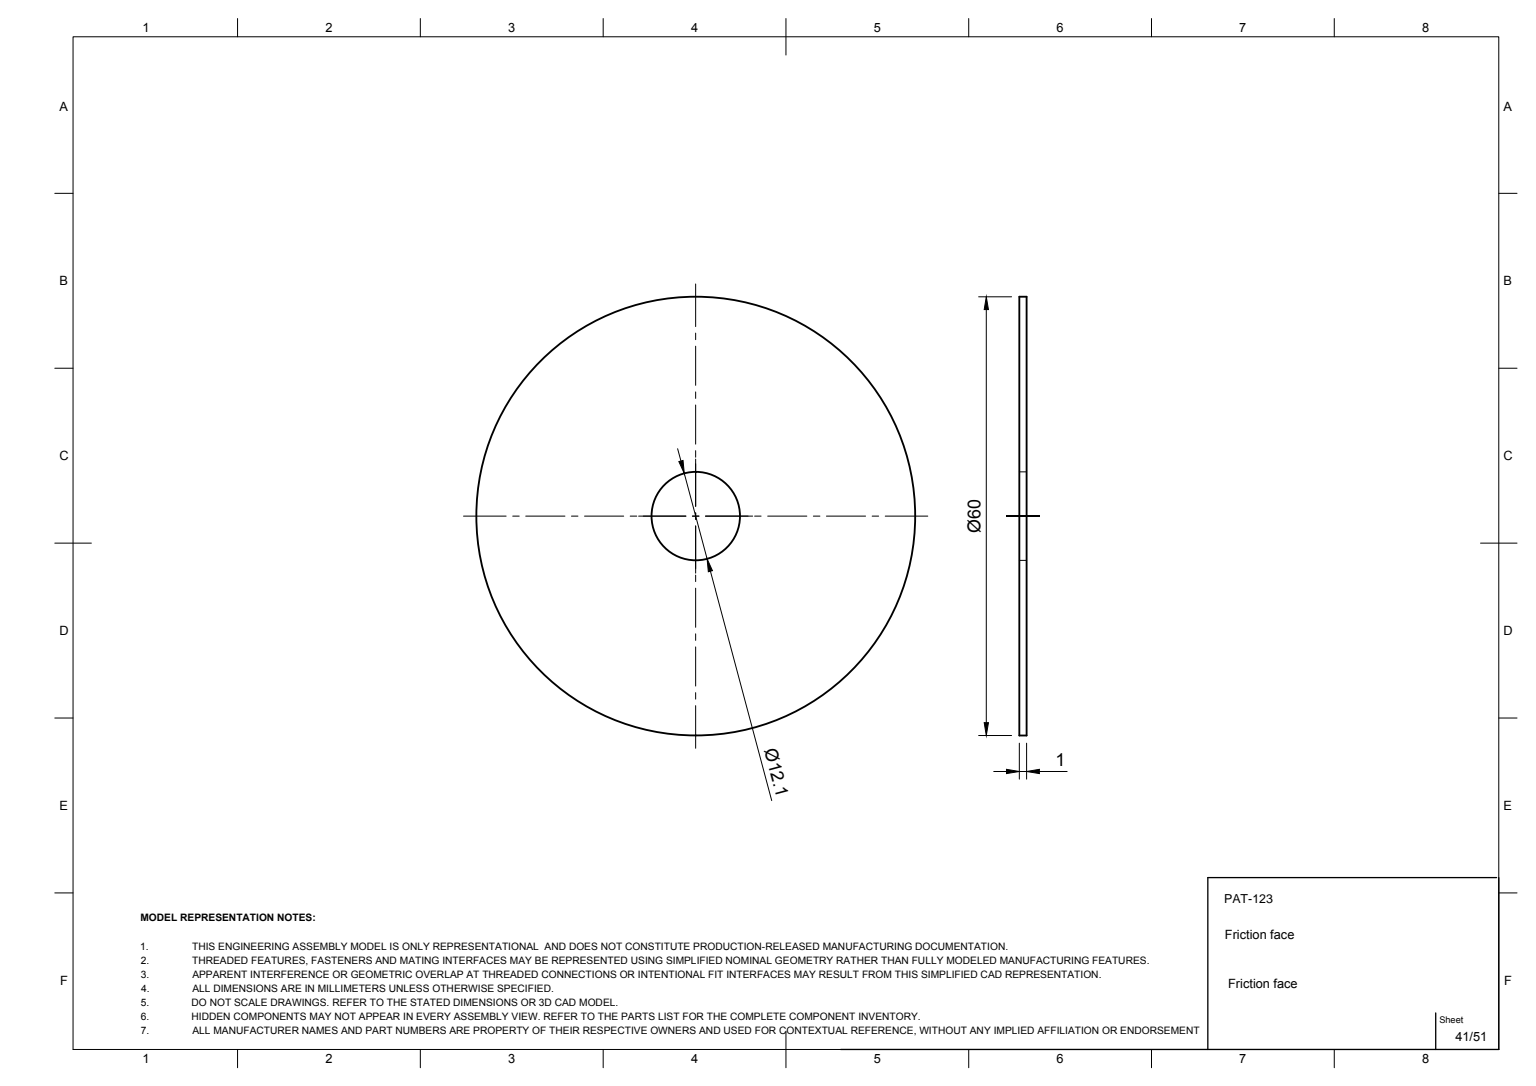
ISO-10303-21;
HEADER;
/* Generated by software containing ST-Developer
 * from STEP Tools, Inc. (www.steptools.com) 
 */

FILE_DESCRIPTION(
/* description */ ('Worm-less right-angle friction wheel drive'),
/* implementation_level */ '2;1');

FILE_NAME(
/* name */ 'Friction face.step',
/* time_stamp */ '2026-10-28T03:22:36-07:00',
/* author */ (''),
/* organization */ (''),
/* preprocessor_version */ 'ST-DEVELOPER v20.2',
/* originating_system */ 'Autodesk Translation Framework v15.17.0.0',
/* authorisation */ '');

FILE_SCHEMA (('AUTOMOTIVE_DESIGN { 1 0 10303 214 3 1 1 }'));
ENDSEC;

DATA;
#10=MECHANICAL_DESIGN_GEOMETRIC_PRESENTATION_REPRESENTATION('',(#654),#17046);
#553=SHAPE_REPRESENTATION_RELATIONSHIP('SRR','None',#17298,#600);
#600=ADVANCED_BREP_SHAPE_REPRESENTATION('',(#705),#17034);
#654=STYLED_ITEM('',(#17577),#705);
#705=MANIFOLD_SOLID_BREP('Body1',#8212);
#932=FACE_BOUND('',#2271,.T.);
#933=FACE_BOUND('',#2273,.T.);
#1147=PLANE('',#9528);
#1148=PLANE('',#9529);
#1585=FACE_OUTER_BOUND('',#2268,.T.);
#1586=FACE_OUTER_BOUND('',#2269,.T.);
#1587=FACE_OUTER_BOUND('',#2270,.T.);
#1588=FACE_OUTER_BOUND('',#2272,.T.);
#2268=EDGE_LOOP('',(#7166,#7167,#7168,#7169));
#2269=EDGE_LOOP('',(#7170,#7171,#7172,#7173));
#2270=EDGE_LOOP('',(#7174));
#2271=EDGE_LOOP('',(#7175));
#2272=EDGE_LOOP('',(#7176));
#2273=EDGE_LOOP('',(#7177));
#2802=LINE('',#16336,#3342);
#2803=LINE('',#16342,#3343);
#3342=VECTOR('',#11762,0.605);
#3343=VECTOR('',#11769,3.);
#3816=CIRCLE('',#9523,0.605);
#3817=CIRCLE('',#9524,0.605);
#3818=CIRCLE('',#9526,3.);
#3819=CIRCLE('',#9527,3.);
#4417=VERTEX_POINT('',#16333);
#4418=VERTEX_POINT('',#16335);
#4419=VERTEX_POINT('',#16339);
#4420=VERTEX_POINT('',#16341);
#5352=EDGE_CURVE('',#4417,#4417,#3816,.T.);
#5353=EDGE_CURVE('',#4417,#4418,#2802,.T.);
#5354=EDGE_CURVE('',#4418,#4418,#3817,.T.);
#5355=EDGE_CURVE('',#4419,#4419,#3818,.T.);
#5356=EDGE_CURVE('',#4419,#4420,#2803,.T.);
#5357=EDGE_CURVE('',#4420,#4420,#3819,.T.);
#7166=ORIENTED_EDGE('',*,*,#5352,.F.);
#7167=ORIENTED_EDGE('',*,*,#5353,.T.);
#7168=ORIENTED_EDGE('',*,*,#5354,.T.);
#7169=ORIENTED_EDGE('',*,*,#5353,.F.);
#7170=ORIENTED_EDGE('',*,*,#5355,.F.);
#7171=ORIENTED_EDGE('',*,*,#5356,.T.);
#7172=ORIENTED_EDGE('',*,*,#5357,.T.);
#7173=ORIENTED_EDGE('',*,*,#5356,.F.);
#7174=ORIENTED_EDGE('',*,*,#5355,.T.);
#7175=ORIENTED_EDGE('',*,*,#5352,.T.);
#7176=ORIENTED_EDGE('',*,*,#5357,.F.);
#7177=ORIENTED_EDGE('',*,*,#5354,.F.);
#7677=CYLINDRICAL_SURFACE('',#9522,0.605);
#7678=CYLINDRICAL_SURFACE('',#9525,3.);
#8077=ADVANCED_FACE('',(#1585),#7677,.F.);
#8078=ADVANCED_FACE('',(#1586),#7678,.T.);
#8079=ADVANCED_FACE('',(#1587,#932),#1147,.T.);
#8080=ADVANCED_FACE('',(#1588,#933),#1148,.F.);
#8212=CLOSED_SHELL('',(#8077,#8078,#8079,#8080));
#9521=AXIS2_PLACEMENT_3D('',#16331,#11756,#11757);
#9522=AXIS2_PLACEMENT_3D('',#16332,#11758,#11759);
#9523=AXIS2_PLACEMENT_3D('',#16334,#11760,#11761);
#9524=AXIS2_PLACEMENT_3D('',#16337,#11763,#11764);
#9525=AXIS2_PLACEMENT_3D('',#16338,#11765,#11766);
#9526=AXIS2_PLACEMENT_3D('',#16340,#11767,#11768);
#9527=AXIS2_PLACEMENT_3D('',#16343,#11770,#11771);
#9528=AXIS2_PLACEMENT_3D('',#16344,#11772,#11773);
#9529=AXIS2_PLACEMENT_3D('',#16345,#11774,#11775);
#11756=DIRECTION('axis',(0.,0.,1.));
#11757=DIRECTION('refdir',(1.,0.,0.));
#11758=DIRECTION('center_axis',(0.,1.,0.));
#11759=DIRECTION('ref_axis',(1.,0.,0.));
#11760=DIRECTION('center_axis',(0.,-1.,0.));
#11761=DIRECTION('ref_axis',(1.,0.,0.));
#11762=DIRECTION('',(0.,-1.,0.));
#11763=DIRECTION('center_axis',(0.,-1.,0.));
#11764=DIRECTION('ref_axis',(1.,0.,0.));
#11765=DIRECTION('center_axis',(0.,1.,0.));
#11766=DIRECTION('ref_axis',(1.,0.,0.));
#11767=DIRECTION('center_axis',(0.,1.,0.));
#11768=DIRECTION('ref_axis',(1.,0.,0.));
#11769=DIRECTION('',(0.,-1.,0.));
#11770=DIRECTION('center_axis',(0.,1.,0.));
#11771=DIRECTION('ref_axis',(1.,0.,0.));
#11772=DIRECTION('center_axis',(0.,1.,0.));
#11773=DIRECTION('ref_axis',(1.,0.,0.));
#11774=DIRECTION('center_axis',(0.,1.,0.));
#11775=DIRECTION('ref_axis',(1.,0.,0.));
#16331=CARTESIAN_POINT('',(0.,0.,0.));
#16332=CARTESIAN_POINT('Origin',(0.,-0.1,7.));
#16333=CARTESIAN_POINT('',(-0.605,0.,7.));
#16334=CARTESIAN_POINT('Origin',(0.,0.,7.));
#16335=CARTESIAN_POINT('',(-0.605,-0.1,7.));
#16336=CARTESIAN_POINT('',(-0.605,-0.1,7.));
#16337=CARTESIAN_POINT('Origin',(0.,-0.1,7.));
#16338=CARTESIAN_POINT('Origin',(0.,-0.1,7.));
#16339=CARTESIAN_POINT('',(-3.,0.,7.));
#16340=CARTESIAN_POINT('Origin',(0.,0.,7.));
#16341=CARTESIAN_POINT('',(-3.,-0.1,7.));
#16342=CARTESIAN_POINT('',(-3.,-0.1,7.));
#16343=CARTESIAN_POINT('Origin',(0.,-0.1,7.));
#16344=CARTESIAN_POINT('Origin',(0.,0.,7.));
#16345=CARTESIAN_POINT('Origin',(0.,-0.1,7.));
#16981=UNCERTAINTY_MEASURE_WITH_UNIT(LENGTH_MEASURE(0.001),#17047,
'DISTANCE_ACCURACY_VALUE',
'Maximum model space distance between geometric entities at asserted c
onnectivities');
#16993=UNCERTAINTY_MEASURE_WITH_UNIT(LENGTH_MEASURE(0.001),#17047,
'DISTANCE_ACCURACY_VALUE',
'Maximum model space distance between geometric entities at asserted c
onnectivities');
#17034=(
GEOMETRIC_REPRESENTATION_CONTEXT(3)
GLOBAL_UNCERTAINTY_ASSIGNED_CONTEXT((#16981))
GLOBAL_UNIT_ASSIGNED_CONTEXT((#17047,#17049,#17050))
REPRESENTATION_CONTEXT('','3D')
);
#17046=(
GEOMETRIC_REPRESENTATION_CONTEXT(3)
GLOBAL_UNCERTAINTY_ASSIGNED_CONTEXT((#16993))
GLOBAL_UNIT_ASSIGNED_CONTEXT((#17047,#17049,#17050))
REPRESENTATION_CONTEXT('','3D')
);
#17047=(
LENGTH_UNIT()
NAMED_UNIT(*)
SI_UNIT(.CENTI.,.METRE.)
);
#17049=(
NAMED_UNIT(*)
PLANE_ANGLE_UNIT()
SI_UNIT($,.RADIAN.)
);
#17050=(
NAMED_UNIT(*)
SI_UNIT($,.STERADIAN.)
SOLID_ANGLE_UNIT()
);
#17091=SHAPE_DEFINITION_REPRESENTATION(#17148,#17298);
#17148=PRODUCT_DEFINITION_SHAPE('',$,#17351);
#17298=SHAPE_REPRESENTATION('',(#9521),#17034);
#17310=PRODUCT_DEFINITION_CONTEXT('part definition',#17468,'design');
#17351=PRODUCT_DEFINITION('Friction face','Friction face',#17403,#17310);
#17403=PRODUCT_DEFINITION_FORMATION('',$,#17510);
#17468=APPLICATION_CONTEXT(
'Core Data for Automotive Mechanical Design Process');
#17469=PRODUCT_CONTEXT('part definition',#17468,'mechanical');
#17510=PRODUCT('Friction face','Friction face','Friction face',(#17469));
#17571=COLOUR_RGB('Light Blue',0.38,0.62,0.78);
#17572=FILL_AREA_STYLE_COLOUR('',#17571);
#17573=FILL_AREA_STYLE('',(#17572));
#17574=SURFACE_STYLE_FILL_AREA(#17573);
#17575=SURFACE_SIDE_STYLE('',(#17574));
#17576=SURFACE_STYLE_USAGE(.BOTH.,#17575);
#17577=PRESENTATION_STYLE_ASSIGNMENT((#17576));
ENDSEC;
END-ISO-10303-21;
